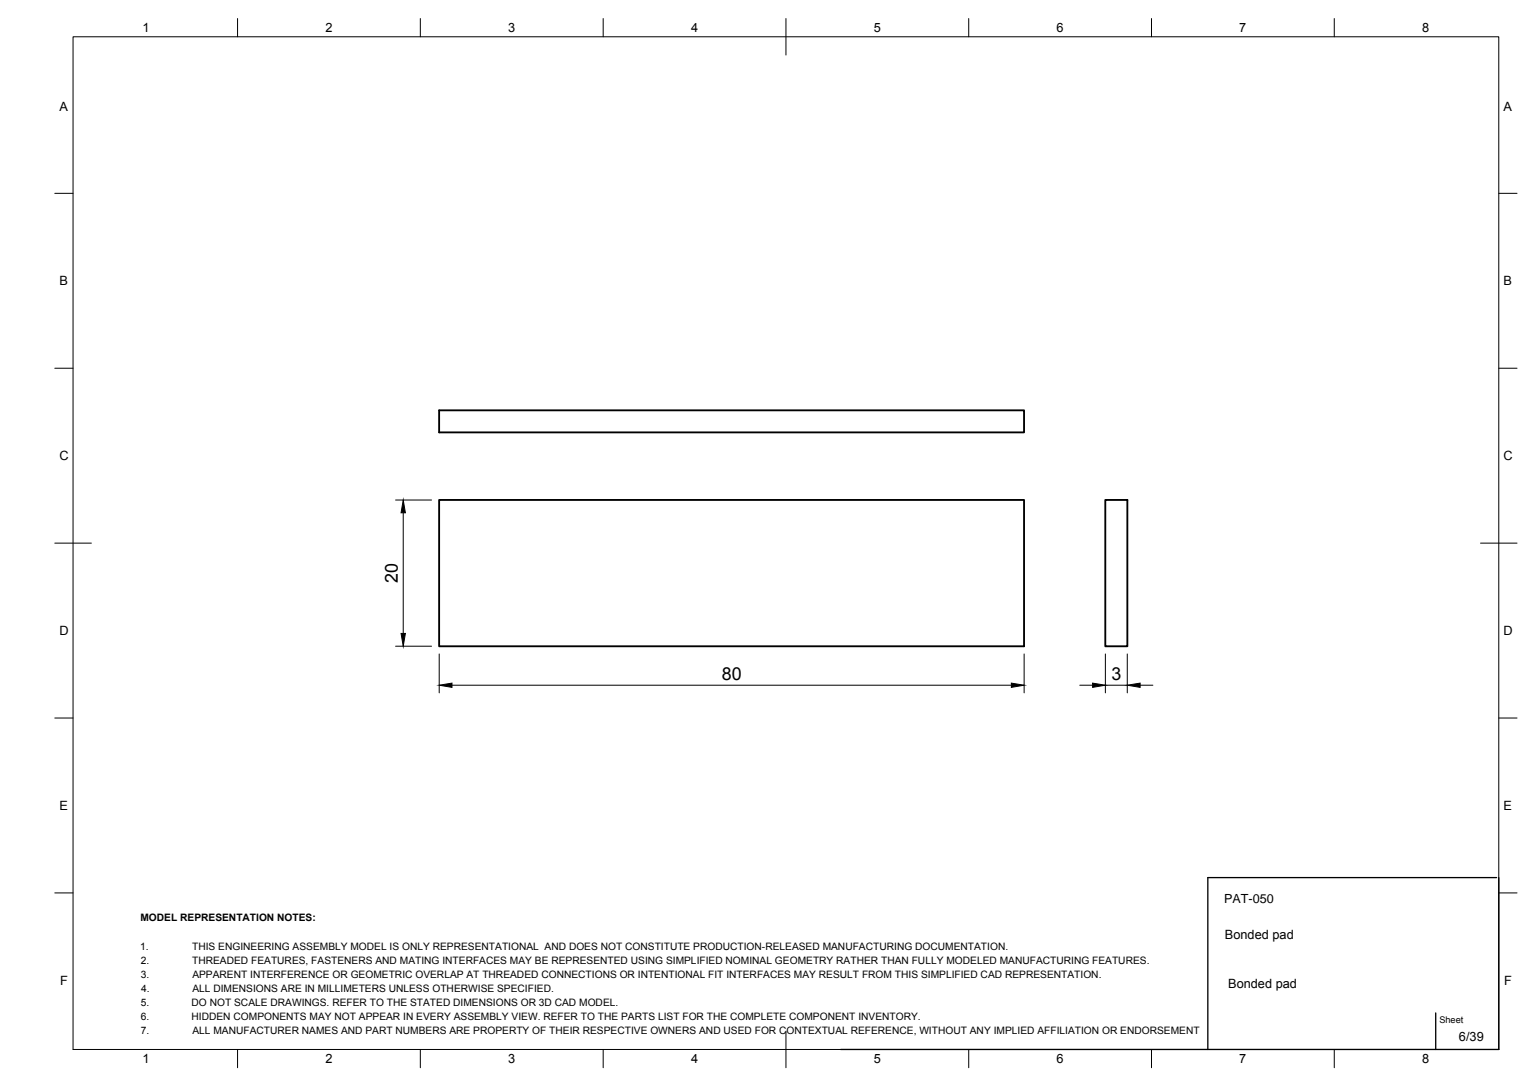
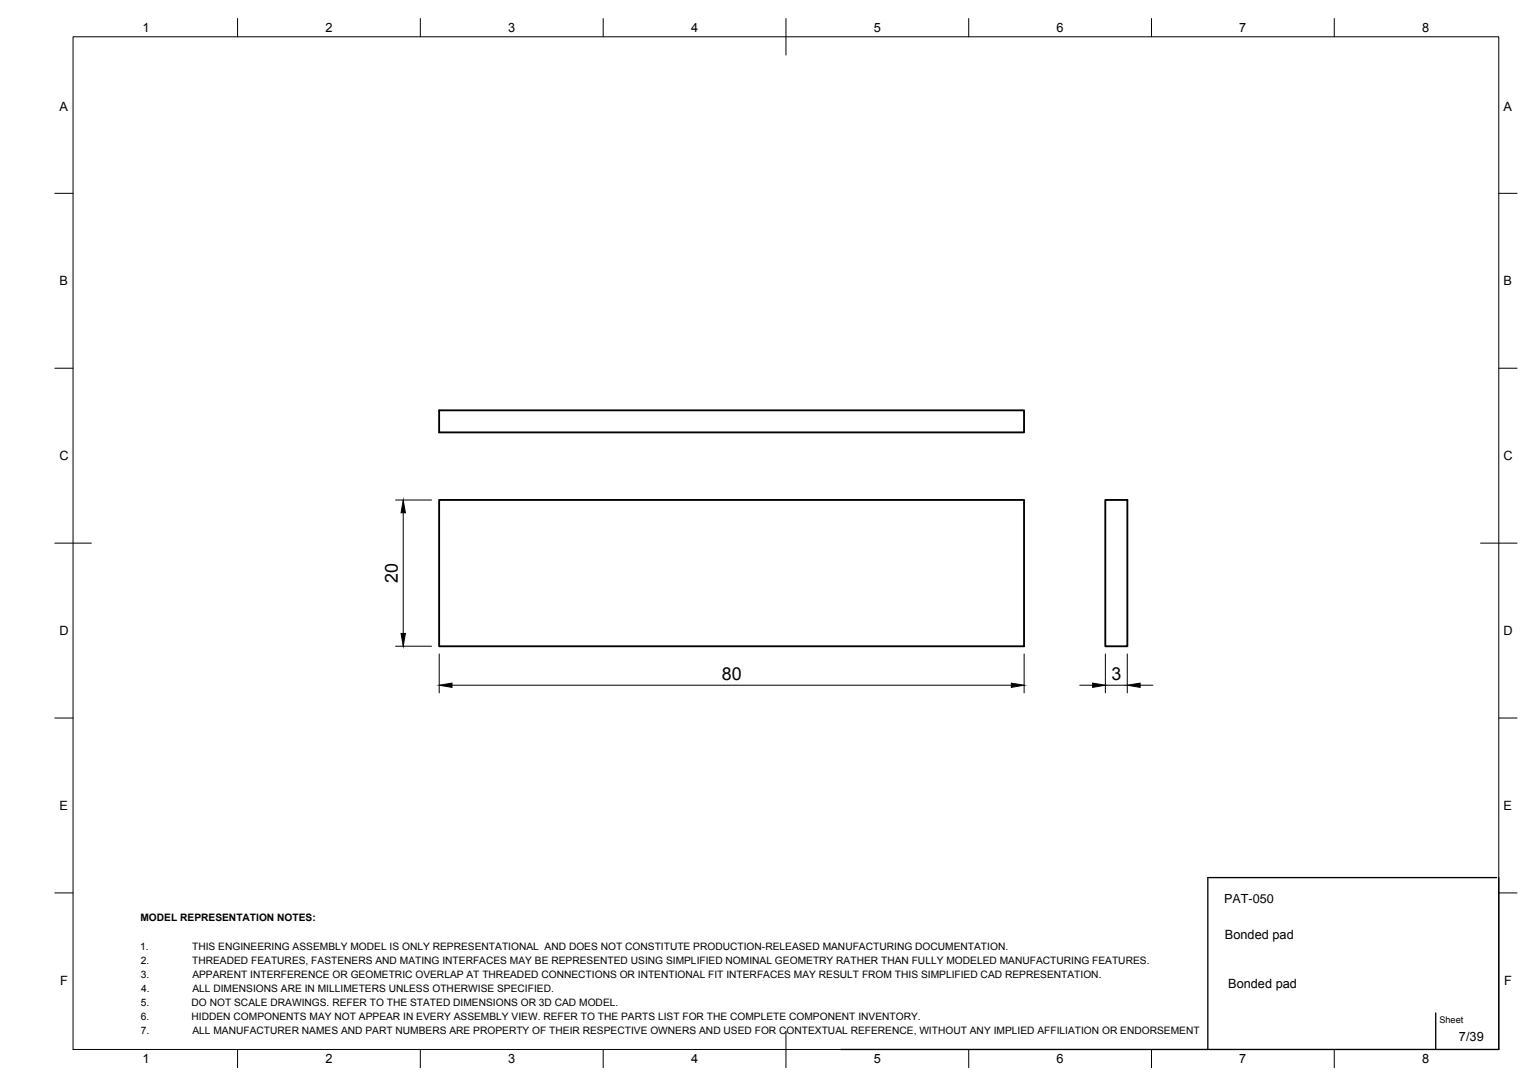
ISO-10303-21;
HEADER;
/* Generated by software containing ST-Developer
 * from STEP Tools, Inc. (www.steptools.com) 
 */

FILE_DESCRIPTION(
/* description */ ('Hand wheel with handle and shaft collar'),
/* implementation_level */ '2;1');

FILE_NAME(
/* name */ 'Bonded pad.step',
/* time_stamp */ '2026-10-28T03:23:19-07:00',
/* author */ (''),
/* organization */ (''),
/* preprocessor_version */ 'ST-DEVELOPER v20.2',
/* originating_system */ 'Autodesk Translation Framework v15.17.0.0',
/* authorisation */ '');

FILE_SCHEMA (('AUTOMOTIVE_DESIGN { 1 0 10303 214 3 1 1 }'));
ENDSEC;

DATA;
#10=MECHANICAL_DESIGN_GEOMETRIC_PRESENTATION_REPRESENTATION('',(#396),#10510);
#332=SHAPE_REPRESENTATION_RELATIONSHIP('SRR','None',#10648,#364);
#364=ADVANCED_BREP_SHAPE_REPRESENTATION('',(#443),#10475);
#396=STYLED_ITEM('',(#10922),#443);
#443=MANIFOLD_SOLID_BREP('Body1',#5295);
#604=PLANE('',#5719);
#605=PLANE('',#5720);
#606=PLANE('',#5721);
#607=PLANE('',#5722);
#608=PLANE('',#5723);
#609=PLANE('',#5724);
#773=FACE_OUTER_BOUND('',#1100,.T.);
#774=FACE_OUTER_BOUND('',#1101,.T.);
#775=FACE_OUTER_BOUND('',#1102,.T.);
#776=FACE_OUTER_BOUND('',#1103,.T.);
#777=FACE_OUTER_BOUND('',#1104,.T.);
#778=FACE_OUTER_BOUND('',#1105,.T.);
#1100=EDGE_LOOP('',(#3605,#3606,#3607,#3608));
#1101=EDGE_LOOP('',(#3609,#3610,#3611,#3612));
#1102=EDGE_LOOP('',(#3613,#3614,#3615,#3616));
#1103=EDGE_LOOP('',(#3617,#3618,#3619,#3620));
#1104=EDGE_LOOP('',(#3621,#3622,#3623,#3624));
#1105=EDGE_LOOP('',(#3625,#3626,#3627,#3628));
#1529=LINE('',#8230,#1839);
#1530=LINE('',#8232,#1840);
#1531=LINE('',#8234,#1841);
#1532=LINE('',#8235,#1842);
#1533=LINE('',#8238,#1843);
#1534=LINE('',#8240,#1844);
#1535=LINE('',#8241,#1845);
#1536=LINE('',#8244,#1846);
#1537=LINE('',#8246,#1847);
#1538=LINE('',#8247,#1848);
#1539=LINE('',#8249,#1849);
#1540=LINE('',#8250,#1850);
#1839=VECTOR('',#6481,1.);
#1840=VECTOR('',#6482,1.);
#1841=VECTOR('',#6483,1.);
#1842=VECTOR('',#6484,1.);
#1843=VECTOR('',#6487,1.);
#1844=VECTOR('',#6488,1.);
#1845=VECTOR('',#6489,1.);
#1846=VECTOR('',#6492,1.);
#1847=VECTOR('',#6493,1.);
#1848=VECTOR('',#6494,1.);
#1849=VECTOR('',#6497,1.);
#1850=VECTOR('',#6498,1.);
#2460=VERTEX_POINT('',#8228);
#2461=VERTEX_POINT('',#8229);
#2462=VERTEX_POINT('',#8231);
#2463=VERTEX_POINT('',#8233);
#2464=VERTEX_POINT('',#8237);
#2465=VERTEX_POINT('',#8239);
#2466=VERTEX_POINT('',#8243);
#2467=VERTEX_POINT('',#8245);
#2920=EDGE_CURVE('',#2460,#2461,#1529,.T.);
#2921=EDGE_CURVE('',#2461,#2462,#1530,.T.);
#2922=EDGE_CURVE('',#2463,#2462,#1531,.T.);
#2923=EDGE_CURVE('',#2460,#2463,#1532,.T.);
#2924=EDGE_CURVE('',#2464,#2460,#1533,.T.);
#2925=EDGE_CURVE('',#2465,#2463,#1534,.T.);
#2926=EDGE_CURVE('',#2464,#2465,#1535,.T.);
#2927=EDGE_CURVE('',#2466,#2464,#1536,.T.);
#2928=EDGE_CURVE('',#2467,#2465,#1537,.T.);
#2929=EDGE_CURVE('',#2466,#2467,#1538,.T.);
#2930=EDGE_CURVE('',#2461,#2466,#1539,.T.);
#2931=EDGE_CURVE('',#2462,#2467,#1540,.T.);
#3605=ORIENTED_EDGE('',*,*,#2920,.T.);
#3606=ORIENTED_EDGE('',*,*,#2921,.T.);
#3607=ORIENTED_EDGE('',*,*,#2922,.F.);
#3608=ORIENTED_EDGE('',*,*,#2923,.F.);
#3609=ORIENTED_EDGE('',*,*,#2924,.T.);
#3610=ORIENTED_EDGE('',*,*,#2923,.T.);
#3611=ORIENTED_EDGE('',*,*,#2925,.F.);
#3612=ORIENTED_EDGE('',*,*,#2926,.F.);
#3613=ORIENTED_EDGE('',*,*,#2927,.T.);
#3614=ORIENTED_EDGE('',*,*,#2926,.T.);
#3615=ORIENTED_EDGE('',*,*,#2928,.F.);
#3616=ORIENTED_EDGE('',*,*,#2929,.F.);
#3617=ORIENTED_EDGE('',*,*,#2930,.T.);
#3618=ORIENTED_EDGE('',*,*,#2929,.T.);
#3619=ORIENTED_EDGE('',*,*,#2931,.F.);
#3620=ORIENTED_EDGE('',*,*,#2921,.F.);
#3621=ORIENTED_EDGE('',*,*,#2931,.T.);
#3622=ORIENTED_EDGE('',*,*,#2928,.T.);
#3623=ORIENTED_EDGE('',*,*,#2925,.T.);
#3624=ORIENTED_EDGE('',*,*,#2922,.T.);
#3625=ORIENTED_EDGE('',*,*,#2930,.F.);
#3626=ORIENTED_EDGE('',*,*,#2920,.F.);
#3627=ORIENTED_EDGE('',*,*,#2924,.F.);
#3628=ORIENTED_EDGE('',*,*,#2927,.F.);
#4985=ADVANCED_FACE('',(#773),#604,.T.);
#4986=ADVANCED_FACE('',(#774),#605,.T.);
#4987=ADVANCED_FACE('',(#775),#606,.T.);
#4988=ADVANCED_FACE('',(#776),#607,.T.);
#4989=ADVANCED_FACE('',(#777),#608,.T.);
#4990=ADVANCED_FACE('',(#778),#609,.F.);
#5295=CLOSED_SHELL('',(#4985,#4986,#4987,#4988,#4989,#4990));
#5718=AXIS2_PLACEMENT_3D('',#8226,#6477,#6478);
#5719=AXIS2_PLACEMENT_3D('',#8227,#6479,#6480);
#5720=AXIS2_PLACEMENT_3D('',#8236,#6485,#6486);
#5721=AXIS2_PLACEMENT_3D('',#8242,#6490,#6491);
#5722=AXIS2_PLACEMENT_3D('',#8248,#6495,#6496);
#5723=AXIS2_PLACEMENT_3D('',#8251,#6499,#6500);
#5724=AXIS2_PLACEMENT_3D('',#8252,#6501,#6502);
#6477=DIRECTION('axis',(0.,0.,1.));
#6478=DIRECTION('refdir',(1.,0.,0.));
#6479=DIRECTION('center_axis',(0.,1.,0.));
#6480=DIRECTION('ref_axis',(-1.,0.,0.));
#6481=DIRECTION('',(-1.,0.,0.));
#6482=DIRECTION('',(0.,0.,1.));
#6483=DIRECTION('',(-1.,0.,0.));
#6484=DIRECTION('',(0.,0.,1.));
#6485=DIRECTION('center_axis',(1.,0.,0.));
#6486=DIRECTION('ref_axis',(0.,1.,0.));
#6487=DIRECTION('',(0.,1.,0.));
#6488=DIRECTION('',(0.,1.,0.));
#6489=DIRECTION('',(0.,0.,1.));
#6490=DIRECTION('center_axis',(0.,-1.,0.));
#6491=DIRECTION('ref_axis',(1.,0.,0.));
#6492=DIRECTION('',(1.,0.,0.));
#6493=DIRECTION('',(1.,0.,0.));
#6494=DIRECTION('',(0.,0.,1.));
#6495=DIRECTION('center_axis',(-1.,0.,0.));
#6496=DIRECTION('ref_axis',(0.,-1.,0.));
#6497=DIRECTION('',(0.,-1.,0.));
#6498=DIRECTION('',(0.,-1.,0.));
#6499=DIRECTION('center_axis',(0.,0.,1.));
#6500=DIRECTION('ref_axis',(1.,0.,0.));
#6501=DIRECTION('center_axis',(0.,0.,1.));
#6502=DIRECTION('ref_axis',(1.,0.,0.));
#8226=CARTESIAN_POINT('',(0.,0.,0.));
#8227=CARTESIAN_POINT('Origin',(-7.5,7.,-0.3));
#8228=CARTESIAN_POINT('',(-7.5,7.,-0.3));
#8229=CARTESIAN_POINT('',(-9.5,7.,-0.3));
#8230=CARTESIAN_POINT('',(-7.5,7.,-0.3));
#8231=CARTESIAN_POINT('',(-9.5,7.,0.));
#8232=CARTESIAN_POINT('',(-9.5,7.,-0.3));
#8233=CARTESIAN_POINT('',(-7.5,7.,0.));
#8234=CARTESIAN_POINT('',(-7.5,7.,0.));
#8235=CARTESIAN_POINT('',(-7.5,7.,-0.3));
#8236=CARTESIAN_POINT('Origin',(-7.5,-1.,-0.3));
#8237=CARTESIAN_POINT('',(-7.5,-1.,-0.3));
#8238=CARTESIAN_POINT('',(-7.5,-1.,-0.3));
#8239=CARTESIAN_POINT('',(-7.5,-1.,0.));
#8240=CARTESIAN_POINT('',(-7.5,-1.,0.));
#8241=CARTESIAN_POINT('',(-7.5,-1.,-0.3));
#8242=CARTESIAN_POINT('Origin',(-9.5,-1.,-0.3));
#8243=CARTESIAN_POINT('',(-9.5,-1.,-0.3));
#8244=CARTESIAN_POINT('',(-9.5,-1.,-0.3));
#8245=CARTESIAN_POINT('',(-9.5,-1.,0.));
#8246=CARTESIAN_POINT('',(-9.5,-1.,0.));
#8247=CARTESIAN_POINT('',(-9.5,-1.,-0.3));
#8248=CARTESIAN_POINT('Origin',(-9.5,7.,-0.3));
#8249=CARTESIAN_POINT('',(-9.5,7.,-0.3));
#8250=CARTESIAN_POINT('',(-9.5,7.,0.));
#8251=CARTESIAN_POINT('Origin',(-8.5,3.,0.));
#8252=CARTESIAN_POINT('Origin',(-8.5,3.,-0.3));
#10436=UNCERTAINTY_MEASURE_WITH_UNIT(LENGTH_MEASURE(0.001),#10511,
'DISTANCE_ACCURACY_VALUE',
'Maximum model space distance between geometric entities at asserted c
onnectivities');
#10471=UNCERTAINTY_MEASURE_WITH_UNIT(LENGTH_MEASURE(0.001),#10511,
'DISTANCE_ACCURACY_VALUE',
'Maximum model space distance between geometric entities at asserted c
onnectivities');
#10475=(
GEOMETRIC_REPRESENTATION_CONTEXT(3)
GLOBAL_UNCERTAINTY_ASSIGNED_CONTEXT((#10436))
GLOBAL_UNIT_ASSIGNED_CONTEXT((#10511,#10513,#10514))
REPRESENTATION_CONTEXT('','3D')
);
#10510=(
GEOMETRIC_REPRESENTATION_CONTEXT(3)
GLOBAL_UNCERTAINTY_ASSIGNED_CONTEXT((#10471))
GLOBAL_UNIT_ASSIGNED_CONTEXT((#10511,#10513,#10514))
REPRESENTATION_CONTEXT('','3D')
);
#10511=(
LENGTH_UNIT()
NAMED_UNIT(*)
SI_UNIT(.CENTI.,.METRE.)
);
#10513=(
NAMED_UNIT(*)
PLANE_ANGLE_UNIT()
SI_UNIT($,.RADIAN.)
);
#10514=(
NAMED_UNIT(*)
SI_UNIT($,.STERADIAN.)
SOLID_ANGLE_UNIT()
);
#10518=SHAPE_DEFINITION_REPRESENTATION(#10556,#10648);
#10556=PRODUCT_DEFINITION_SHAPE('',$,#10687);
#10648=SHAPE_REPRESENTATION('',(#5718),#10475);
#10683=PRODUCT_DEFINITION_CONTEXT('part definition',#10799,'design');
#10687=PRODUCT_DEFINITION('Bonded pad','Bonded pad',#10725,#10683);
#10725=PRODUCT_DEFINITION_FORMATION('',$,#10804);
#10799=APPLICATION_CONTEXT(
'Core Data for Automotive Mechanical Design Process');
#10800=PRODUCT_CONTEXT('part definition',#10799,'mechanical');
#10804=PRODUCT('Bonded pad','Bonded pad','Bonded pad',(#10800));
#10916=COLOUR_RGB('Off White',0.89,0.88,0.83);
#10917=FILL_AREA_STYLE_COLOUR('',#10916);
#10918=FILL_AREA_STYLE('',(#10917));
#10919=SURFACE_STYLE_FILL_AREA(#10918);
#10920=SURFACE_SIDE_STYLE('',(#10919));
#10921=SURFACE_STYLE_USAGE(.BOTH.,#10920);
#10922=PRESENTATION_STYLE_ASSIGNMENT((#10921));
ENDSEC;
END-ISO-10303-21;
